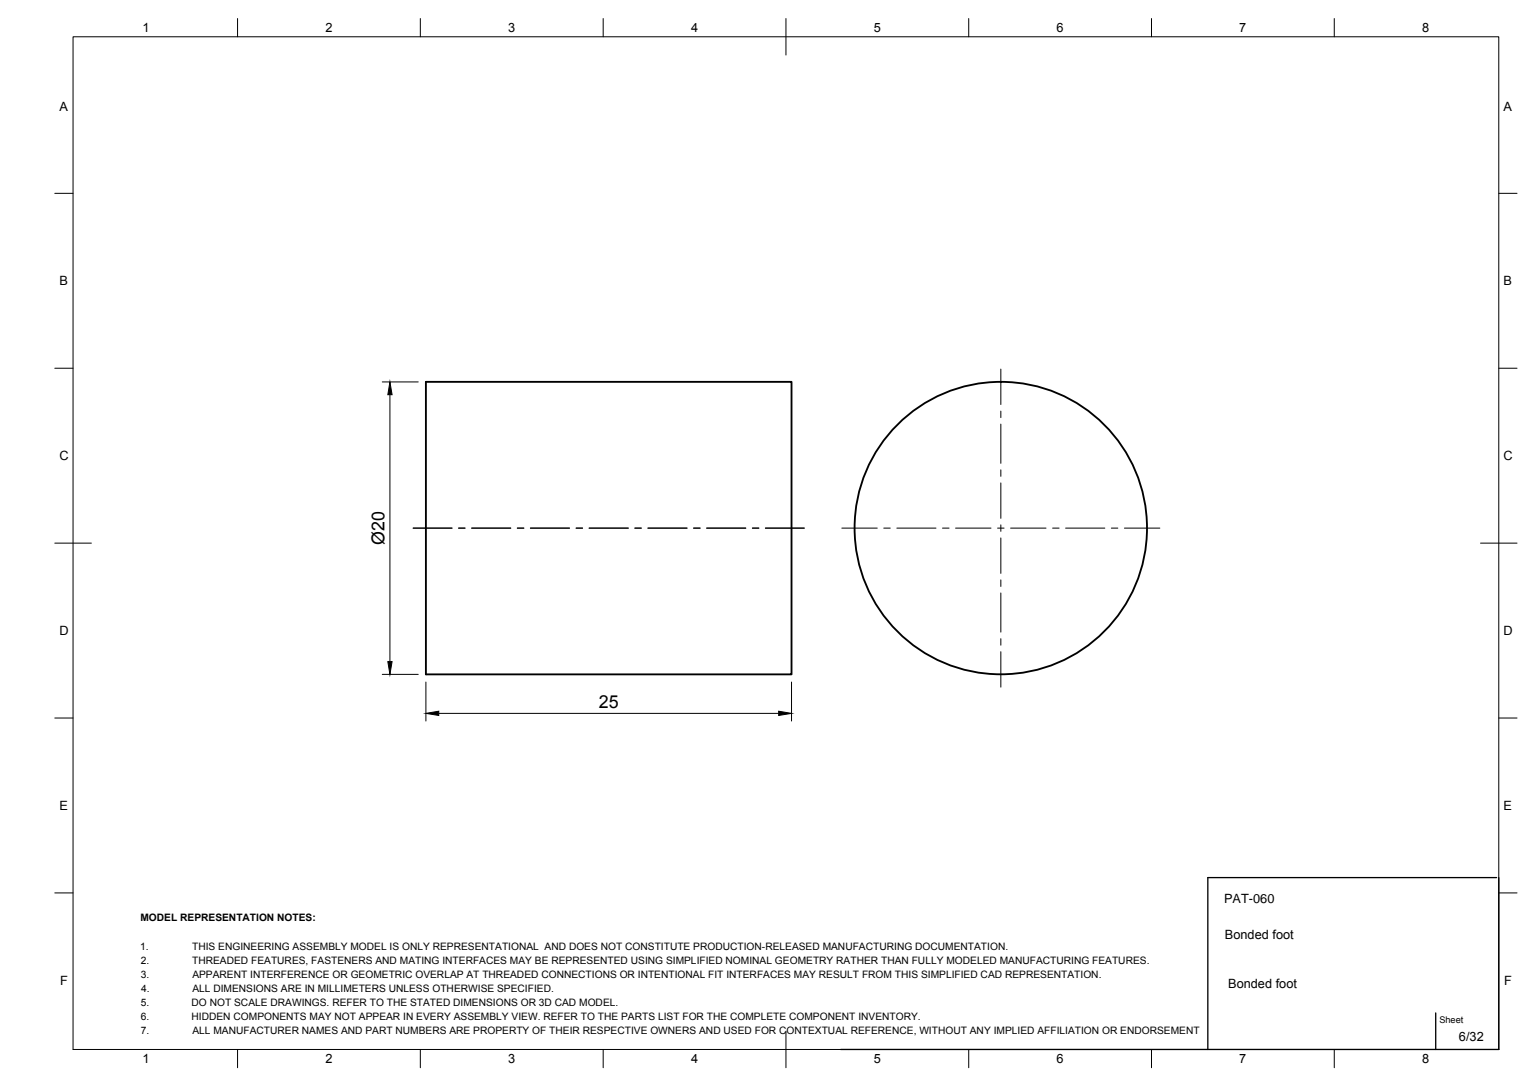
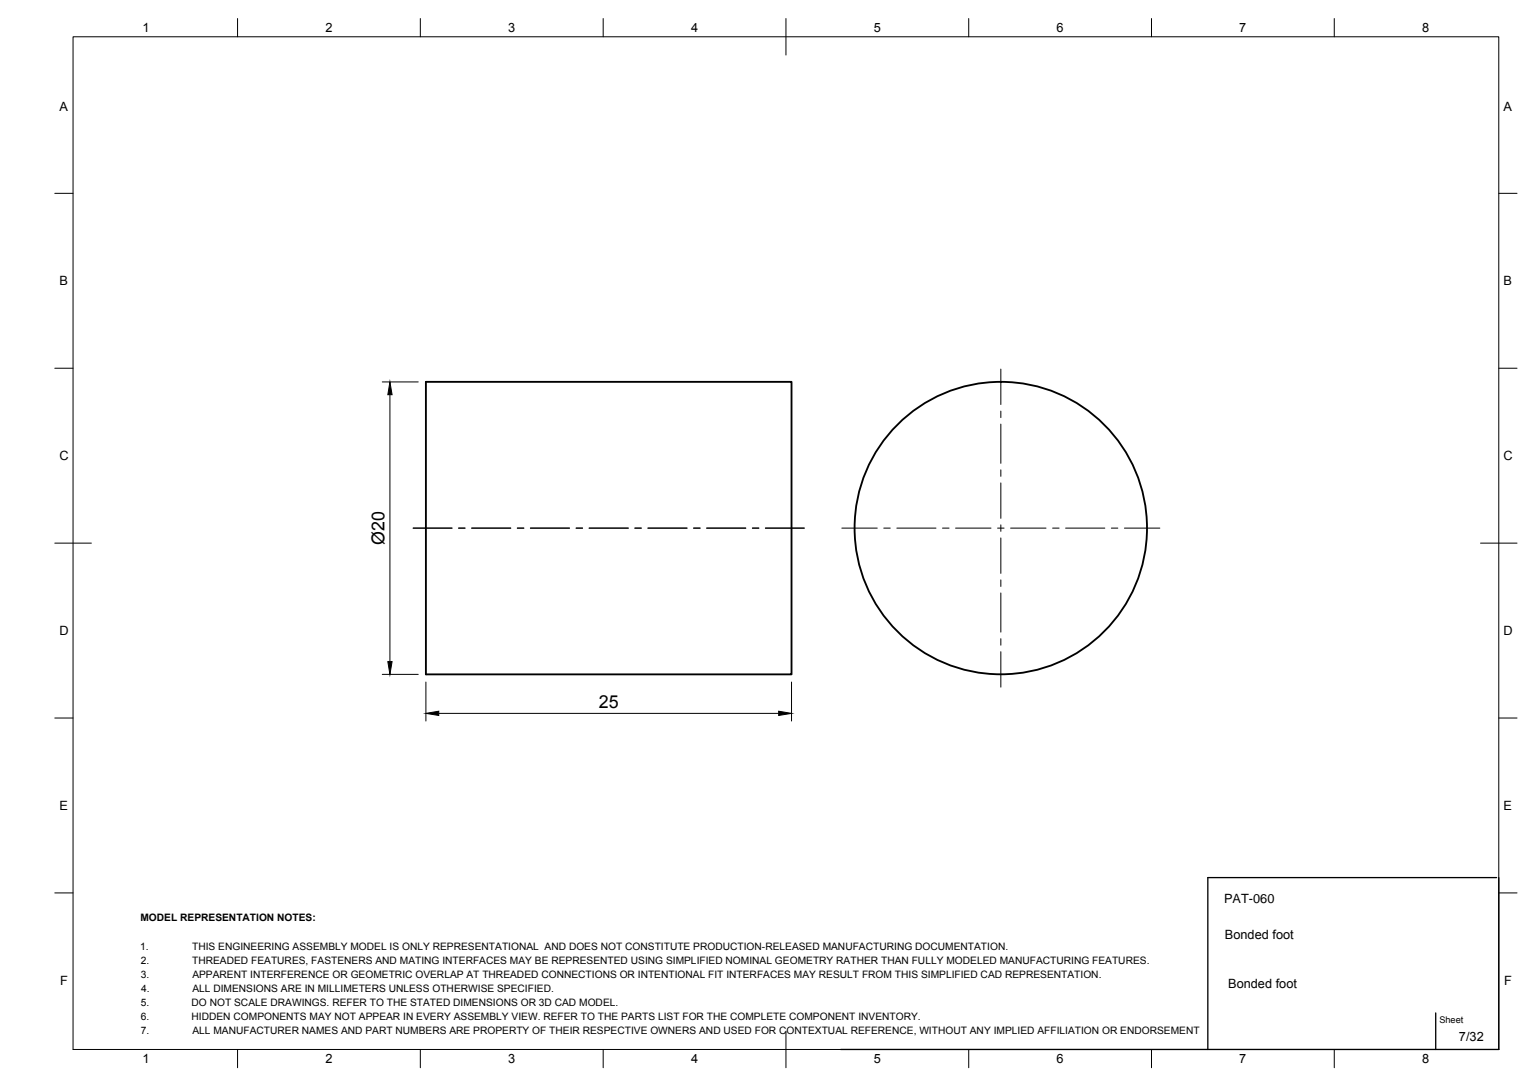
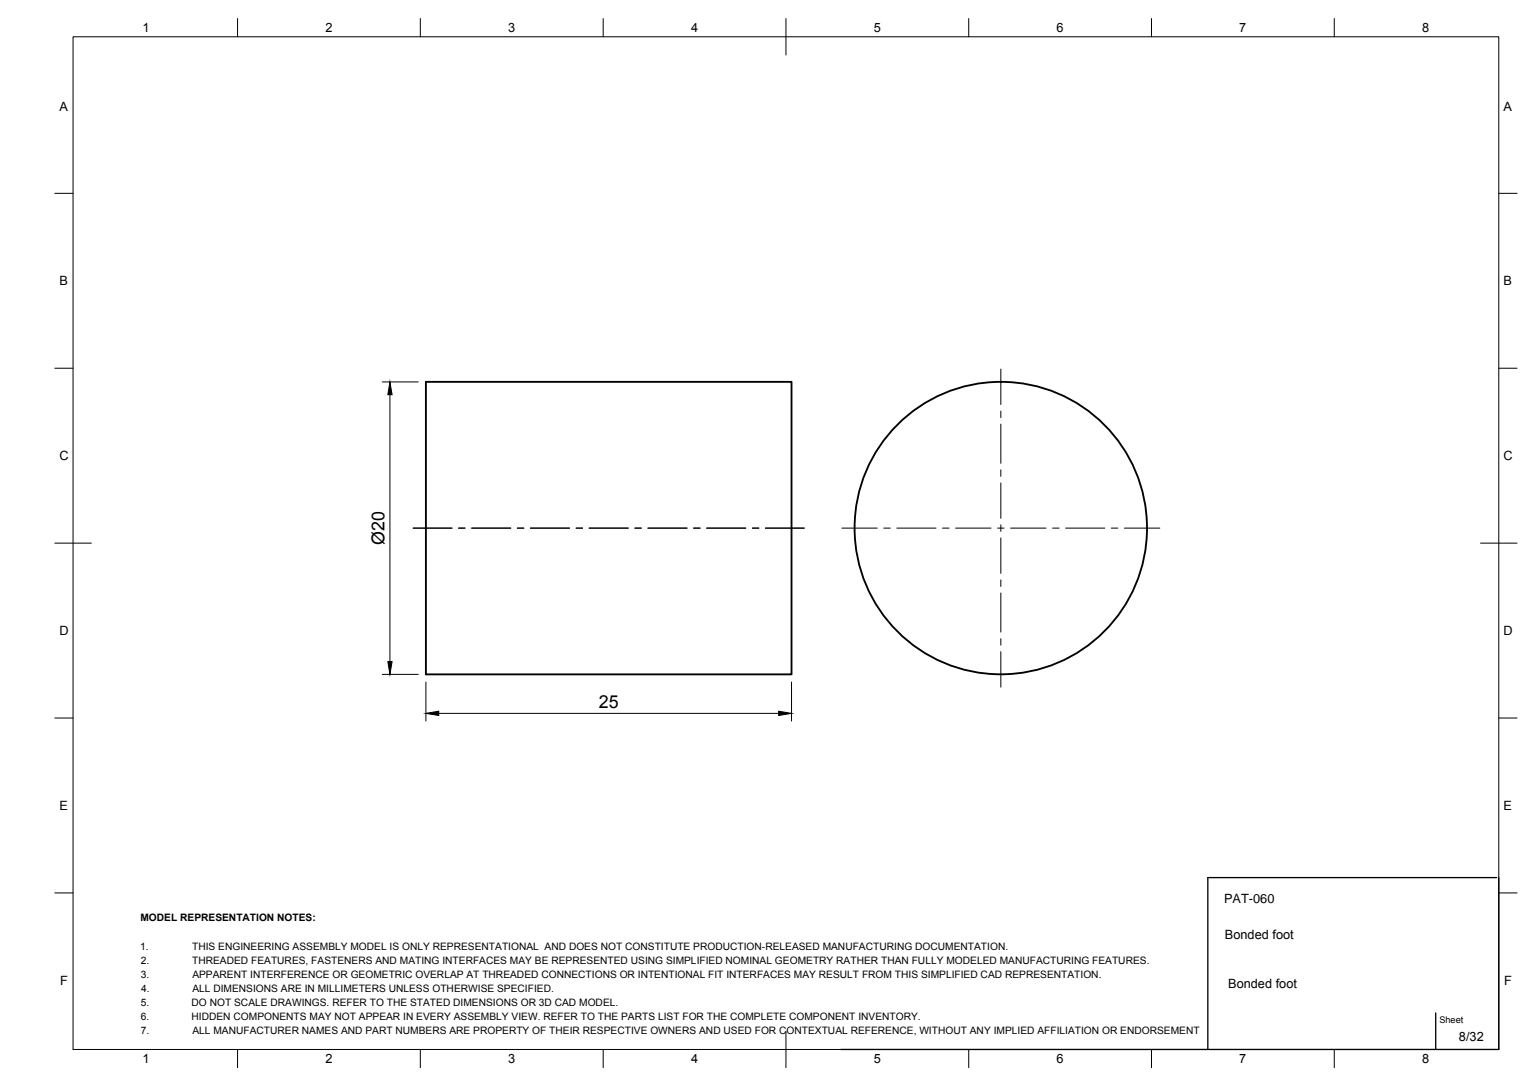
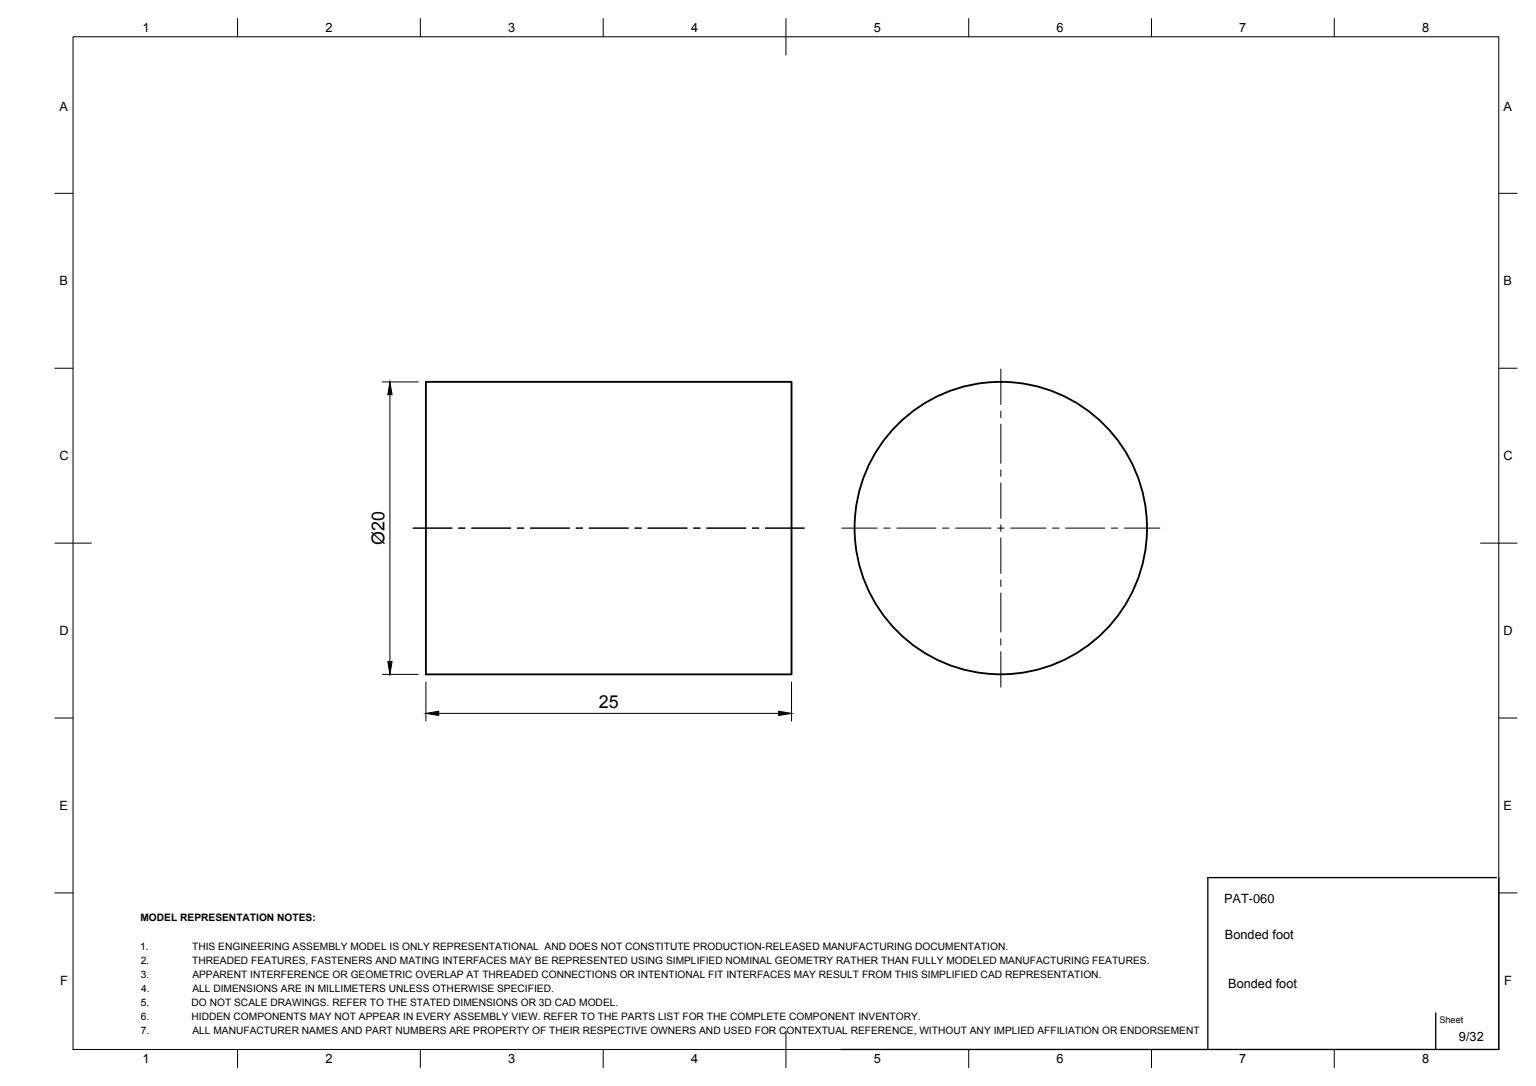
ISO-10303-21;
HEADER;
/* Generated by software containing ST-Developer
 * from STEP Tools, Inc. (www.steptools.com) 
 */

FILE_DESCRIPTION(
/* description */ ('Indexing fixture plate with plunger'),
/* implementation_level */ '2;1');

FILE_NAME(
/* name */ 'Bonded foot.step',
/* time_stamp */ '2026-10-28T03:23:41-07:00',
/* author */ (''),
/* organization */ (''),
/* preprocessor_version */ 'ST-DEVELOPER v20.2',
/* originating_system */ 'Autodesk Translation Framework v15.17.0.0',
/* authorisation */ '');

FILE_SCHEMA (('AUTOMOTIVE_DESIGN { 1 0 10303 214 3 1 1 }'));
ENDSEC;

DATA;
#10=MECHANICAL_DESIGN_GEOMETRIC_PRESENTATION_REPRESENTATION('',(#318),#10020);
#264=SHAPE_REPRESENTATION_RELATIONSHIP('SRR','None',#10138,#291);
#291=ADVANCED_BREP_SHAPE_REPRESENTATION('',(#354),#9991);
#318=STYLED_ITEM('',(#10382),#354);
#354=MANIFOLD_SOLID_BREP('Body1',#4572);
#543=PLANE('',#4941);
#544=PLANE('',#4942);
#683=FACE_OUTER_BOUND('',#983,.T.);
#684=FACE_OUTER_BOUND('',#984,.T.);
#685=FACE_OUTER_BOUND('',#985,.T.);
#983=EDGE_LOOP('',(#3129,#3130,#3131,#3132));
#984=EDGE_LOOP('',(#3133));
#985=EDGE_LOOP('',(#3134));
#1411=LINE('',#7201,#1631);
#1631=VECTOR('',#5658,1.);
#1846=CIRCLE('',#4939,1.);
#1847=CIRCLE('',#4940,1.);
#2157=VERTEX_POINT('',#7198);
#2158=VERTEX_POINT('',#7200);
#2544=EDGE_CURVE('',#2157,#2157,#1846,.T.);
#2545=EDGE_CURVE('',#2157,#2158,#1411,.T.);
#2546=EDGE_CURVE('',#2158,#2158,#1847,.T.);
#3129=ORIENTED_EDGE('',*,*,#2544,.F.);
#3130=ORIENTED_EDGE('',*,*,#2545,.T.);
#3131=ORIENTED_EDGE('',*,*,#2546,.T.);
#3132=ORIENTED_EDGE('',*,*,#2545,.F.);
#3133=ORIENTED_EDGE('',*,*,#2544,.T.);
#3134=ORIENTED_EDGE('',*,*,#2546,.F.);
#4174=CYLINDRICAL_SURFACE('',#4938,1.);
#4298=ADVANCED_FACE('',(#683),#4174,.T.);
#4299=ADVANCED_FACE('',(#684),#543,.T.);
#4300=ADVANCED_FACE('',(#685),#544,.F.);
#4572=CLOSED_SHELL('',(#4298,#4299,#4300));
#4937=AXIS2_PLACEMENT_3D('',#7196,#5652,#5653);
#4938=AXIS2_PLACEMENT_3D('',#7197,#5654,#5655);
#4939=AXIS2_PLACEMENT_3D('',#7199,#5656,#5657);
#4940=AXIS2_PLACEMENT_3D('',#7202,#5659,#5660);
#4941=AXIS2_PLACEMENT_3D('',#7203,#5661,#5662);
#4942=AXIS2_PLACEMENT_3D('',#7204,#5663,#5664);
#5652=DIRECTION('axis',(0.,0.,1.));
#5653=DIRECTION('refdir',(1.,0.,0.));
#5654=DIRECTION('center_axis',(0.,0.,1.));
#5655=DIRECTION('ref_axis',(1.,0.,0.));
#5656=DIRECTION('center_axis',(0.,0.,1.));
#5657=DIRECTION('ref_axis',(1.,0.,0.));
#5658=DIRECTION('',(0.,0.,-1.));
#5659=DIRECTION('center_axis',(0.,0.,1.));
#5660=DIRECTION('ref_axis',(1.,0.,0.));
#5661=DIRECTION('center_axis',(0.,0.,1.));
#5662=DIRECTION('ref_axis',(1.,0.,0.));
#5663=DIRECTION('center_axis',(0.,0.,1.));
#5664=DIRECTION('ref_axis',(1.,0.,0.));
#7196=CARTESIAN_POINT('',(0.,0.,0.));
#7197=CARTESIAN_POINT('Origin',(-9.5,-9.5,-3.5));
#7198=CARTESIAN_POINT('',(-10.5,-9.5,-1.));
#7199=CARTESIAN_POINT('Origin',(-9.5,-9.5,-1.));
#7200=CARTESIAN_POINT('',(-10.5,-9.5,-3.5));
#7201=CARTESIAN_POINT('',(-10.5,-9.5,-3.5));
#7202=CARTESIAN_POINT('Origin',(-9.5,-9.5,-3.5));
#7203=CARTESIAN_POINT('Origin',(-9.5,-9.5,-1.));
#7204=CARTESIAN_POINT('Origin',(-9.5,-9.5,-3.5));
#9958=UNCERTAINTY_MEASURE_WITH_UNIT(LENGTH_MEASURE(0.001),#10021,
'DISTANCE_ACCURACY_VALUE',
'Maximum model space distance between geometric entities at asserted c
onnectivities');
#9987=UNCERTAINTY_MEASURE_WITH_UNIT(LENGTH_MEASURE(0.001),#10021,
'DISTANCE_ACCURACY_VALUE',
'Maximum model space distance between geometric entities at asserted c
onnectivities');
#9991=(
GEOMETRIC_REPRESENTATION_CONTEXT(3)
GLOBAL_UNCERTAINTY_ASSIGNED_CONTEXT((#9958))
GLOBAL_UNIT_ASSIGNED_CONTEXT((#10021,#10023,#10024))
REPRESENTATION_CONTEXT('','3D')
);
#10020=(
GEOMETRIC_REPRESENTATION_CONTEXT(3)
GLOBAL_UNCERTAINTY_ASSIGNED_CONTEXT((#9987))
GLOBAL_UNIT_ASSIGNED_CONTEXT((#10021,#10023,#10024))
REPRESENTATION_CONTEXT('','3D')
);
#10021=(
LENGTH_UNIT()
NAMED_UNIT(*)
SI_UNIT(.CENTI.,.METRE.)
);
#10023=(
NAMED_UNIT(*)
PLANE_ANGLE_UNIT()
SI_UNIT($,.RADIAN.)
);
#10024=(
NAMED_UNIT(*)
SI_UNIT($,.STERADIAN.)
SOLID_ANGLE_UNIT()
);
#10028=SHAPE_DEFINITION_REPRESENTATION(#10060,#10138);
#10060=PRODUCT_DEFINITION_SHAPE('',$,#10171);
#10138=SHAPE_REPRESENTATION('',(#4937),#9991);
#10167=PRODUCT_DEFINITION_CONTEXT('part definition',#10265,'design');
#10171=PRODUCT_DEFINITION('Bonded foot','Bonded foot',#10203,#10167);
#10203=PRODUCT_DEFINITION_FORMATION('',$,#10270);
#10265=APPLICATION_CONTEXT(
'Core Data for Automotive Mechanical Design Process');
#10266=PRODUCT_CONTEXT('part definition',#10265,'mechanical');
#10270=PRODUCT('Bonded foot','Bonded foot','Bonded foot',(#10266));
#10376=COLOUR_RGB('Off White',0.89,0.88,0.83);
#10377=FILL_AREA_STYLE_COLOUR('',#10376);
#10378=FILL_AREA_STYLE('',(#10377));
#10379=SURFACE_STYLE_FILL_AREA(#10378);
#10380=SURFACE_SIDE_STYLE('',(#10379));
#10381=SURFACE_STYLE_USAGE(.BOTH.,#10380);
#10382=PRESENTATION_STYLE_ASSIGNMENT((#10381));
ENDSEC;
END-ISO-10303-21;
